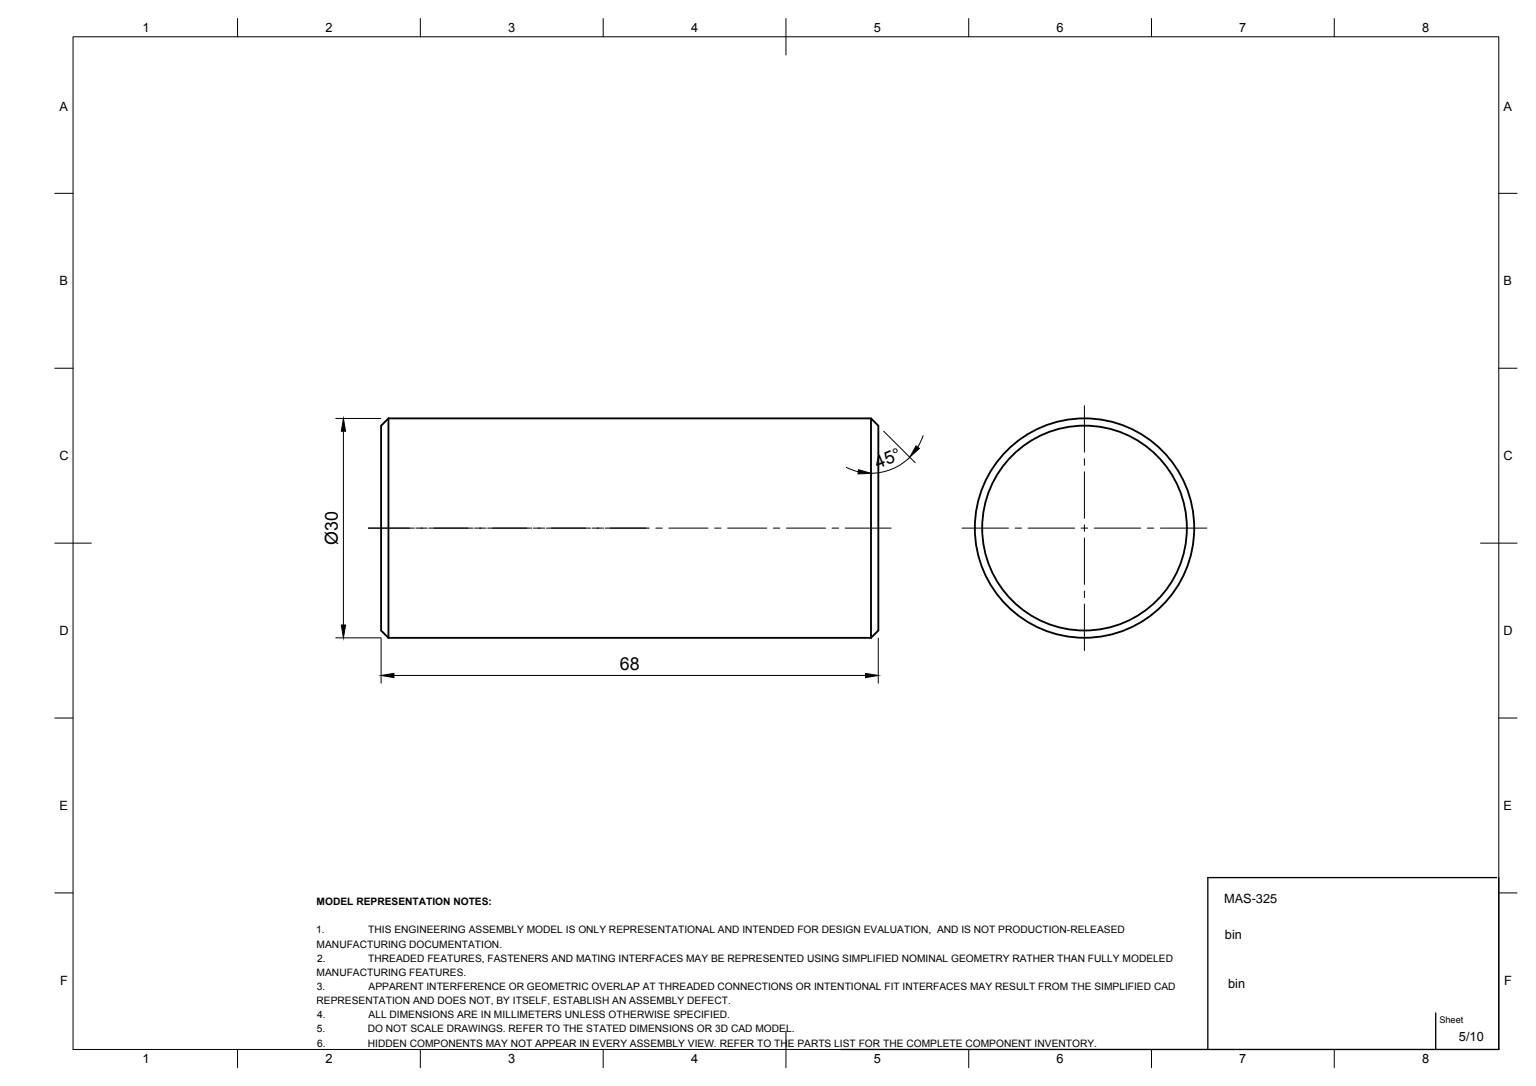
ISO-10303-21;
HEADER;
FILE_DESCRIPTION (('STEP AP214'),
    '1' );
FILE_NAME ('bin.step',
    '2026-10-08T01:23:29',
    ( '' ),
    ( '' ),
    'SwSTEP 2.0',
    'SolidWorks 2025',
    '' );
FILE_SCHEMA (( 'AUTOMOTIVE_DESIGN' ));
ENDSEC;

DATA;
#84=ORIENTED_EDGE ( 'NONE', *, *, #48754, .F. ) ;
#196=AXIS2_PLACEMENT_3D ( 'NONE', #12070, #3180, #43634 ) ;
#279=LINE ( 'NONE', #11844, #1238 ) ;
#1066=CIRCLE ( 'NONE', #196, 14.00000000000001066 ) ;
#1238=VECTOR ( 'NONE', #39954, 1000.000000000000000 ) ;
#1819=DIRECTION ( 'NONE',  ( -0.000000000000000000, 1.000000000000000000, -0.000000000000000000 ) ) ;
#1961=CARTESIAN_POINT ( 'NONE',  ( -48.47912675150885065, -187.5000000000000284, 6.938893903907228378E-15 ) ) ;
#2083=PRODUCT_DEFINITION_SHAPE ( 'NONE', 'NONE',  #38299 ) ;
#2517=DIRECTION ( 'NONE',  ( 0.000000000000000000, -1.000000000000000000, 0.000000000000000000 ) ) ;
#3046=AXIS2_PLACEMENT_3D ( 'NONE', #50143, #42223, #22005 ) ;
#3059=AXIS2_PLACEMENT_3D ( 'NONE', #27944, #4046, #12435 ) ;
#3180=DIRECTION ( 'NONE',  ( 0.000000000000000000, 1.000000000000000000, 0.000000000000000000 ) ) ;
#3242=PRODUCT_DEFINITION_FORMATION_WITH_SPECIFIED_SOURCE ( 'ANY', '', #30214, .NOT_KNOWN. ) ;
#3603=CARTESIAN_POINT ( 'NONE',  ( -48.47912675150885065, -121.5000000000000142, -14.99999999999999289 ) ) ;
#3714=CARTESIAN_POINT ( 'NONE',  ( 0.000000000000000000, 0.000000000000000000, 0.000000000000000000 ) ) ;
#3778=VERTEX_POINT ( 'NONE', #29899 ) ;
#4046=DIRECTION ( 'NONE',  ( 0.000000000000000000, -1.000000000000000000, 0.000000000000000000 ) ) ;
#4510=( NAMED_UNIT ( * ) PLANE_ANGLE_UNIT ( ) SI_UNIT ( $, .RADIAN. ) );
#4771=SURFACE_STYLE_FILL_AREA ( #16612 ) ;
#4897=CIRCLE ( 'NONE', #30885, 13.99999999999998934 ) ;
#5795=CARTESIAN_POINT ( 'NONE',  ( -48.47912675150885065, -187.5000000000000284, 6.938893903907228378E-15 ) ) ;
#6271=LINE ( 'NONE', #34879, #19847 ) ;
#6477=FACE_OUTER_BOUND ( 'NONE', #9992, .T. ) ;
#6647=CARTESIAN_POINT ( 'NONE',  ( -48.47912675150885065, -188.5000000000000284, -13.99999999999998224 ) ) ;
#6811=EDGE_LOOP ( 'NONE', ( #10708, #40354, #10931, #11264 ) ) ;
#6851=CARTESIAN_POINT ( 'NONE',  ( -48.47912675150885065, -120.5000000000000284, 6.938893903907228378E-15 ) ) ;
#6873=CARTESIAN_POINT ( 'NONE',  ( -48.47912675150885065, -188.5000000000000284, 6.938893903907228378E-15 ) ) ;
#7690=AXIS2_PLACEMENT_3D ( 'NONE', #6873, #31035, #19227 ) ;
#7721=EDGE_LOOP ( 'NONE', ( #49434, #14352, #28270, #36379 ) ) ;
#7914=( NAMED_UNIT ( * ) SI_UNIT ( $, .STERADIAN. ) SOLID_ANGLE_UNIT ( ) );
#8105=CARTESIAN_POINT ( 'NONE',  ( -48.47912675150885065, -188.5000000000000284, 6.938893903907228378E-15 ) ) ;
#8183=APPLICATION_CONTEXT ( 'automotive_design' ) ;
#8286=CARTESIAN_POINT ( 'NONE',  ( -48.47912675150885065, -120.5000000000000284, 6.938893903907228378E-15 ) ) ;
#8438=DIRECTION ( 'NONE',  ( 1.000000000000000000, 0.000000000000000000, 0.000000000000000000 ) ) ;
#8761=VERTEX_POINT ( 'NONE', #3603 ) ;
#9079=CARTESIAN_POINT ( 'NONE',  ( -48.47912675150885065, -188.5000000000000284, 13.99999999999999645 ) ) ;
#9244=CARTESIAN_POINT ( 'NONE',  ( -48.47912675150885065, -187.5000000000000284, 6.938893903907228378E-15 ) ) ;
#9754=SHAPE_REPRESENTATION_RELATIONSHIP ( 'NONE' , 'NONE' ,  #33452, #24902 ) ;
#9854=VERTEX_POINT ( 'NONE', #6647 ) ;
#9992=EDGE_LOOP ( 'NONE', ( #19717, #11128, #43821, #46814 ) ) ;
#10472=EDGE_CURVE ( 'NONE', #48687, #8761, #10687, .T. ) ;
#10595=DIRECTION ( 'NONE',  ( 0.000000000000000000, 0.7071067811865444641, 0.7071067811865505703 ) ) ;
#10608=ADVANCED_FACE ( 'NONE', ( #51542 ), #12361, .T. ) ;
#10687=CIRCLE ( 'NONE', #16587, 15.00000000000000000 ) ;
#10708=ORIENTED_EDGE ( 'NONE', *, *, #33374, .T. ) ;
#10841=DIRECTION ( 'NONE',  ( -0.000000000000000000, -1.000000000000000000, -0.000000000000000000 ) ) ;
#10931=ORIENTED_EDGE ( 'NONE', *, *, #38993, .T. ) ;
#11056=ADVANCED_FACE ( 'NONE', ( #48050 ), #44103, .F. ) ;
#11128=ORIENTED_EDGE ( 'NONE', *, *, #11873, .F. ) ;
#11264=ORIENTED_EDGE ( 'NONE', *, *, #47091, .F. ) ;
#11269=ORIENTED_EDGE ( 'NONE', *, *, #39480, .T. ) ;
#11502=( GEOMETRIC_REPRESENTATION_CONTEXT ( 3 ) GLOBAL_UNCERTAINTY_ASSIGNED_CONTEXT ( ( #18520 ) ) GLOBAL_UNIT_ASSIGNED_CONTEXT ( ( #27883, #43922, #7914 ) ) REPRESENTATION_CONTEXT ( 'NONE', 'WORKASPACE' ) );
#11582=AXIS2_PLACEMENT_3D ( 'NONE', #8105, #24149, #44381 ) ;
#11844=CARTESIAN_POINT ( 'NONE',  ( -48.47912675150885065, -120.5000000000000284, -14.99999999999999289 ) ) ;
#11873=EDGE_CURVE ( 'NONE', #28415, #12983, #35137, .T. ) ;
#12070=CARTESIAN_POINT ( 'NONE',  ( -48.47912675150885065, -120.5000000000000284, 6.938893903907228378E-15 ) ) ;
#12158=CARTESIAN_POINT ( 'NONE',  ( -48.47912675150885065, -120.5000000000000284, 15.00000000000000711 ) ) ;
#12315=CARTESIAN_POINT ( 'NONE',  ( -48.47912675150885065, -121.5000000000000142, 15.00000000000000711 ) ) ;
#12361=CYLINDRICAL_SURFACE ( 'NONE', #14075, 15.00000000000000000 ) ;
#12435=DIRECTION ( 'NONE',  ( 0.000000000000000000, 0.000000000000000000, -1.000000000000000000 ) ) ;
#12901=PRESENTATION_STYLE_ASSIGNMENT (( #33133 ) ) ;
#12983=VERTEX_POINT ( 'NONE', #20376 ) ;
#13022=VECTOR ( 'NONE', #36703, 999.9999999999998863 ) ;
#13265=ORIENTED_EDGE ( 'NONE', *, *, #52011, .F. ) ;
#13400=FACE_OUTER_BOUND ( 'NONE', #7721, .T. ) ;
#13515=AXIS2_PLACEMENT_3D ( 'NONE', #1961, #34014, #29023 ) ;
#13524=EDGE_LOOP ( 'NONE', ( #13265, #33337, #16856, #41689 ) ) ;
#14037=STYLED_ITEM ( 'NONE', ( #12901 ), #18528 ) ;
#14075=AXIS2_PLACEMENT_3D ( 'NONE', #28117, #19722, #35755 ) ;
#14286=LINE ( 'NONE', #33982, #13022 ) ;
#14352=ORIENTED_EDGE ( 'NONE', *, *, #39480, .F. ) ;
#16090=EDGE_CURVE ( 'NONE', #48687, #3778, #20060, .T. ) ;
#16587=AXIS2_PLACEMENT_3D ( 'NONE', #39191, #26587, #50268 ) ;
#16612=FILL_AREA_STYLE ('',( #41021 ) ) ;
#16856=ORIENTED_EDGE ( 'NONE', *, *, #38993, .F. ) ;
#17678=VECTOR ( 'NONE', #10595, 1000.000000000000000 ) ;
#17823=ORIENTED_EDGE ( 'NONE', *, *, #28134, .F. ) ;
#17903=DIRECTION ( 'NONE',  ( -0.000000000000000000, 1.000000000000000000, -0.000000000000000000 ) ) ;
#18326=( GEOMETRIC_REPRESENTATION_CONTEXT ( 3 ) GLOBAL_UNCERTAINTY_ASSIGNED_CONTEXT ( ( #47410 ) ) GLOBAL_UNIT_ASSIGNED_CONTEXT ( ( #36292, #4510, #27641 ) ) REPRESENTATION_CONTEXT ( 'NONE', 'WORKASPACE' ) );
#18520=UNCERTAINTY_MEASURE_WITH_UNIT (LENGTH_MEASURE( 1.000000000000000082E-05 ), #27883, 'distance_accuracy_value', 'NONE');
#18528=MANIFOLD_SOLID_BREP ( 'Chamfer2', #37139 ) ;
#18539=CIRCLE ( 'NONE', #13515, 15.00000000000000000 ) ;
#18655=ORIENTED_EDGE ( 'NONE', *, *, #47091, .T. ) ;
#18727=CARTESIAN_POINT ( 'NONE',  ( -48.47912675150885065, -188.5000000000000284, 6.938893903907228378E-15 ) ) ;
#18936=CYLINDRICAL_SURFACE ( 'NONE', #33285, 15.00000000000000000 ) ;
#19227=DIRECTION ( 'NONE',  ( 0.000000000000000000, 0.000000000000000000, 1.000000000000000000 ) ) ;
#19402=ORIENTED_EDGE ( 'NONE', *, *, #52011, .T. ) ;
#19544=PRODUCT_DEFINITION_CONTEXT ( 'detailed design', #8183, 'design' ) ;
#19717=ORIENTED_EDGE ( 'NONE', *, *, #32004, .F. ) ;
#19722=DIRECTION ( 'NONE',  ( -0.000000000000000000, -1.000000000000000000, -0.000000000000000000 ) ) ;
#19847=VECTOR ( 'NONE', #22289, 1000.000000000000000 ) ;
#19969=FACE_OUTER_BOUND ( 'NONE', #13524, .T. ) ;
#20060=LINE ( 'NONE', #12158, #29768 ) ;
#20224=DIRECTION ( 'NONE',  ( -0.000000000000000000, 1.000000000000000000, -0.000000000000000000 ) ) ;
#20376=CARTESIAN_POINT ( 'NONE',  ( -48.47912675150885065, -120.5000000000000284, 14.00000000000001776 ) ) ;
#20501=ADVANCED_FACE ( 'NONE', ( #32404 ), #20695, .T. ) ;
#20695=CONICAL_SURFACE ( 'NONE', #3059, 14.00000000000001066, 0.7853981633974491672 ) ;
#21312=APPLICATION_CONTEXT ( 'automotive_design' ) ;
#22005=DIRECTION ( 'NONE',  ( 0.000000000000000000, 0.000000000000000000, 1.000000000000000000 ) ) ;
#22289=DIRECTION ( 'NONE',  ( 8.659560562354969836E-17, 0.7071067811865444641, -0.7071067811865505703 ) ) ;
#22381=ORIENTED_EDGE ( 'NONE', *, *, #45856, .T. ) ;
#23146=DIRECTION ( 'NONE',  ( 0.000000000000000000, 0.000000000000000000, -1.000000000000000000 ) ) ;
#23264=ORIENTED_EDGE ( 'NONE', *, *, #16090, .F. ) ;
#24149=DIRECTION ( 'NONE',  ( 0.000000000000000000, 1.000000000000000000, 0.000000000000000000 ) ) ;
#24344=DIRECTION ( 'NONE',  ( 0.000000000000000000, 1.000000000000000000, 0.000000000000000000 ) ) ;
#24766=VECTOR ( 'NONE', #36767, 999.9999999999998863 ) ;
#24800=ORIENTED_EDGE ( 'NONE', *, *, #33374, .F. ) ;
#24829=DIRECTION ( 'NONE',  ( 0.000000000000000000, -0.000000000000000000, 1.000000000000000000 ) ) ;
#24902=ADVANCED_BREP_SHAPE_REPRESENTATION ( '', ( #18528, #31742 ), #18326 ) ;
#25134=CARTESIAN_POINT ( 'NONE',  ( -48.47912675150885065, -120.5000000000000284, 6.938893903907228378E-15 ) ) ;
#25460=SHAPE_DEFINITION_REPRESENTATION ( #2083, #33452 ) ;
#25722=EDGE_CURVE ( 'NONE', #38994, #3778, #42902, .T. ) ;
#25948=EDGE_LOOP ( 'NONE', ( #17823, #47497, #24800, #84 ) ) ;
#26482=VERTEX_POINT ( 'NONE', #49134 ) ;
#26587=DIRECTION ( 'NONE',  ( 0.000000000000000000, -1.000000000000000000, 0.000000000000000000 ) ) ;
#26819=AXIS2_PLACEMENT_3D ( 'NONE', #8286, #47723, #24829 ) ;
#26855=DIRECTION ( 'NONE',  ( 0.000000000000000000, 0.000000000000000000, 1.000000000000000000 ) ) ;
#27447=MECHANICAL_DESIGN_GEOMETRIC_PRESENTATION_REPRESENTATION('',(#14037),#11502);
#27641=( NAMED_UNIT ( * ) SI_UNIT ( $, .STERADIAN. ) SOLID_ANGLE_UNIT ( ) );
#27725=FACE_OUTER_BOUND ( 'NONE', #46985, .T. ) ;
#27883=( LENGTH_UNIT ( ) NAMED_UNIT ( * ) SI_UNIT ( .MILLI., .METRE. ) );
#27944=CARTESIAN_POINT ( 'NONE',  ( -48.47912675150885065, -120.5000000000000284, 6.938893903907228378E-15 ) ) ;
#28117=CARTESIAN_POINT ( 'NONE',  ( -48.47912675150885065, -120.5000000000000284, 6.938893903907228378E-15 ) ) ;
#28134=EDGE_CURVE ( 'NONE', #12983, #28415, #1066, .T. ) ;
#28270=ORIENTED_EDGE ( 'NONE', *, *, #25722, .T. ) ;
#28415=VERTEX_POINT ( 'NONE', #33750 ) ;
#29023=DIRECTION ( 'NONE',  ( 0.000000000000000000, 0.000000000000000000, 1.000000000000000000 ) ) ;
#29068=ORIENTED_EDGE ( 'NONE', *, *, #11873, .T. ) ;
#29132=PRODUCT_CONTEXT ( 'NONE', #21312, 'mechanical' ) ;
#29340=EDGE_LOOP ( 'NONE', ( #23264, #36181, #18655, #22381 ) ) ;
#29713=DIRECTION ( 'NONE',  ( 0.000000000000000000, 0.000000000000000000, 1.000000000000000000 ) ) ;
#29768=VECTOR ( 'NONE', #40273, 1000.000000000000000 ) ;
#29899=CARTESIAN_POINT ( 'NONE',  ( -48.47912675150885065, -187.5000000000000284, 15.00000000000000711 ) ) ;
#30214=PRODUCT ( 'bin', 'bin', '', ( #29132 ) ) ;
#30445=DIRECTION ( 'NONE',  ( 0.000000000000000000, 0.000000000000000000, 1.000000000000000000 ) ) ;
#30470=AXIS2_PLACEMENT_3D ( 'NONE', #9244, #17903, #29713 ) ;
#30885=AXIS2_PLACEMENT_3D ( 'NONE', #18727, #10841, #26855 ) ;
#31035=DIRECTION ( 'NONE',  ( -0.000000000000000000, -1.000000000000000000, -0.000000000000000000 ) ) ;
#31649=COLOUR_RGB ( '', 0.40784314, 0.44705882, 0.49803922) ;
#31742=AXIS2_PLACEMENT_3D ( 'NONE', #3714, #31843, #8438 ) ;
#31843=DIRECTION ( 'NONE',  ( 0.000000000000000000, 0.000000000000000000, 1.000000000000000000 ) ) ;
#32004=EDGE_CURVE ( 'NONE', #12983, #48687, #14286, .T. ) ;
#32404=FACE_OUTER_BOUND ( 'NONE', #25948, .T. ) ;
#32710=ADVANCED_FACE ( 'NONE', ( #19969 ), #41607, .T. ) ;
#32814=CARTESIAN_POINT ( 'NONE',  ( -48.47912675150885065, -120.5000000000000284, -14.00000000000000355 ) ) ;
#33133=SURFACE_STYLE_USAGE ( .BOTH. , #36043 ) ;
#33244=CONICAL_SURFACE ( 'NONE', #40846, 14.00000000000001066, 0.7853981633974491672 ) ;
#33285=AXIS2_PLACEMENT_3D ( 'NONE', #6851, #34952, #23146 ) ;
#33337=ORIENTED_EDGE ( 'NONE', *, *, #50112, .T. ) ;
#33374=EDGE_CURVE ( 'NONE', #8761, #48687, #34923, .T. ) ;
#33452=SHAPE_REPRESENTATION ( 'bin', ( #31742 ), #18326 ) ;
#33750=CARTESIAN_POINT ( 'NONE',  ( -48.47912675150885065, -120.5000000000000284, -14.00000000000000355 ) ) ;
#33982=CARTESIAN_POINT ( 'NONE',  ( -48.47912675150885065, -120.5000000000000284, 14.00000000000001776 ) ) ;
#34014=DIRECTION ( 'NONE',  ( -0.000000000000000000, 1.000000000000000000, -0.000000000000000000 ) ) ;
#34561=DIRECTION ( 'NONE',  ( 0.000000000000000000, 0.000000000000000000, -1.000000000000000000 ) ) ;
#34879=CARTESIAN_POINT ( 'NONE',  ( -48.47912675150885065, -187.5000000000000284, -14.99999999999999289 ) ) ;
#34923=CIRCLE ( 'NONE', #3046, 15.00000000000000000 ) ;
#34952=DIRECTION ( 'NONE',  ( -0.000000000000000000, -1.000000000000000000, -0.000000000000000000 ) ) ;
#35137=CIRCLE ( 'NONE', #41861, 14.00000000000001066 ) ;
#35727=DIRECTION ( 'NONE',  ( 0.000000000000000000, 0.000000000000000000, 1.000000000000000000 ) ) ;
#35755=DIRECTION ( 'NONE',  ( 0.000000000000000000, 0.000000000000000000, -1.000000000000000000 ) ) ;
#36043=SURFACE_SIDE_STYLE ('',( #4771 ) ) ;
#36181=ORIENTED_EDGE ( 'NONE', *, *, #10472, .T. ) ;
#36292=( LENGTH_UNIT ( ) NAMED_UNIT ( * ) SI_UNIT ( .MILLI., .METRE. ) );
#36379=ORIENTED_EDGE ( 'NONE', *, *, #45856, .F. ) ;
#36703=DIRECTION ( 'NONE',  ( 8.659560562354941486E-17, -0.7071067811865469066, 0.7071067811865482389 ) ) ;
#36767=DIRECTION ( 'NONE',  ( 0.000000000000000000, -0.7071067811865469066, -0.7071067811865482389 ) ) ;
#37139=CLOSED_SHELL ( 'NONE', ( #20501, #32710, #10608, #50897, #37645, #11056, #38169, #50549 ) ) ;
#37190=CIRCLE ( 'NONE', #30470, 15.00000000000000000 ) ;
#37541=LINE ( 'NONE', #32814, #24766 ) ;
#37645=ADVANCED_FACE ( 'NONE', ( #27725 ), #47970, .T. ) ;
#37739=CARTESIAN_POINT ( 'NONE',  ( -48.47912675150885065, -120.5000000000000284, 6.938893903907228378E-15 ) ) ;
#38169=ADVANCED_FACE ( 'NONE', ( #13400 ), #41153, .T. ) ;
#38299=PRODUCT_DEFINITION ( 'UNKNOWN', '', #3242, #19544 ) ;
#38993=EDGE_CURVE ( 'NONE', #3778, #26482, #18539, .T. ) ;
#38994=VERTEX_POINT ( 'NONE', #9079 ) ;
#39191=CARTESIAN_POINT ( 'NONE',  ( -48.47912675150885065, -121.5000000000000142, 6.938893903907228378E-15 ) ) ;
#39480=EDGE_CURVE ( 'NONE', #38994, #9854, #40424, .T. ) ;
#39954=DIRECTION ( 'NONE',  ( -0.000000000000000000, -1.000000000000000000, -0.000000000000000000 ) ) ;
#40273=DIRECTION ( 'NONE',  ( -0.000000000000000000, -1.000000000000000000, -0.000000000000000000 ) ) ;
#40354=ORIENTED_EDGE ( 'NONE', *, *, #16090, .T. ) ;
#40424=CIRCLE ( 'NONE', #7690, 13.99999999999998934 ) ;
#40438=CARTESIAN_POINT ( 'NONE',  ( -48.47912675150885065, -187.5000000000000284, 6.938893903907228378E-15 ) ) ;
#40846=AXIS2_PLACEMENT_3D ( 'NONE', #37739, #2517, #34561 ) ;
#41021=FILL_AREA_STYLE_COLOUR ( '', #31649 ) ;
#41153=CONICAL_SURFACE ( 'NONE', #46201, 15.00000000000000000, 0.7853981633974526089 ) ;
#41607=CONICAL_SURFACE ( 'NONE', #50896, 15.00000000000000000, 0.7853981633974526089 ) ;
#41689=ORIENTED_EDGE ( 'NONE', *, *, #25722, .F. ) ;
#41861=AXIS2_PLACEMENT_3D ( 'NONE', #25134, #24344, #44574 ) ;
#42223=DIRECTION ( 'NONE',  ( 0.000000000000000000, -1.000000000000000000, 0.000000000000000000 ) ) ;
#42902=LINE ( 'NONE', #50298, #17678 ) ;
#43634=DIRECTION ( 'NONE',  ( 0.000000000000000000, 0.000000000000000000, 1.000000000000000000 ) ) ;
#43821=ORIENTED_EDGE ( 'NONE', *, *, #48754, .T. ) ;
#43922=( NAMED_UNIT ( * ) PLANE_ANGLE_UNIT ( ) SI_UNIT ( $, .RADIAN. ) );
#44103=PLANE ( 'NONE',  #11582 ) ;
#44381=DIRECTION ( 'NONE',  ( 0.000000000000000000, -0.000000000000000000, 1.000000000000000000 ) ) ;
#44574=DIRECTION ( 'NONE',  ( 0.000000000000000000, 0.000000000000000000, 1.000000000000000000 ) ) ;
#45152=EDGE_LOOP ( 'NONE', ( #11269, #19402 ) ) ;
#45856=EDGE_CURVE ( 'NONE', #26482, #3778, #37190, .T. ) ;
#45861=ORIENTED_EDGE ( 'NONE', *, *, #28134, .T. ) ;
#46201=AXIS2_PLACEMENT_3D ( 'NONE', #5795, #1819, #30445 ) ;
#46814=ORIENTED_EDGE ( 'NONE', *, *, #10472, .F. ) ;
#46985=EDGE_LOOP ( 'NONE', ( #29068, #45861 ) ) ;
#47091=EDGE_CURVE ( 'NONE', #8761, #26482, #279, .T. ) ;
#47410=UNCERTAINTY_MEASURE_WITH_UNIT (LENGTH_MEASURE( 1.000000000000000082E-05 ), #36292, 'distance_accuracy_value', 'NONE');
#47497=ORIENTED_EDGE ( 'NONE', *, *, #32004, .T. ) ;
#47723=DIRECTION ( 'NONE',  ( 0.000000000000000000, 1.000000000000000000, 0.000000000000000000 ) ) ;
#47970=PLANE ( 'NONE',  #26819 ) ;
#48050=FACE_OUTER_BOUND ( 'NONE', #45152, .T. ) ;
#48687=VERTEX_POINT ( 'NONE', #12315 ) ;
#48754=EDGE_CURVE ( 'NONE', #28415, #8761, #37541, .T. ) ;
#49134=CARTESIAN_POINT ( 'NONE',  ( -48.47912675150885065, -187.5000000000000284, -14.99999999999999289 ) ) ;
#49434=ORIENTED_EDGE ( 'NONE', *, *, #50112, .F. ) ;
#50037=FACE_OUTER_BOUND ( 'NONE', #29340, .T. ) ;
#50112=EDGE_CURVE ( 'NONE', #9854, #26482, #6271, .T. ) ;
#50143=CARTESIAN_POINT ( 'NONE',  ( -48.47912675150885065, -121.5000000000000142, 6.938893903907228378E-15 ) ) ;
#50268=DIRECTION ( 'NONE',  ( 0.000000000000000000, 0.000000000000000000, 1.000000000000000000 ) ) ;
#50298=CARTESIAN_POINT ( 'NONE',  ( -48.47912675150885065, -187.5000000000000284, 15.00000000000000711 ) ) ;
#50549=ADVANCED_FACE ( 'NONE', ( #6477 ), #33244, .T. ) ;
#50896=AXIS2_PLACEMENT_3D ( 'NONE', #40438, #20224, #35727 ) ;
#50897=ADVANCED_FACE ( 'NONE', ( #50037 ), #18936, .T. ) ;
#51542=FACE_OUTER_BOUND ( 'NONE', #6811, .T. ) ;
#52011=EDGE_CURVE ( 'NONE', #9854, #38994, #4897, .T. ) ;
ENDSEC;
END-ISO-10303-21;
